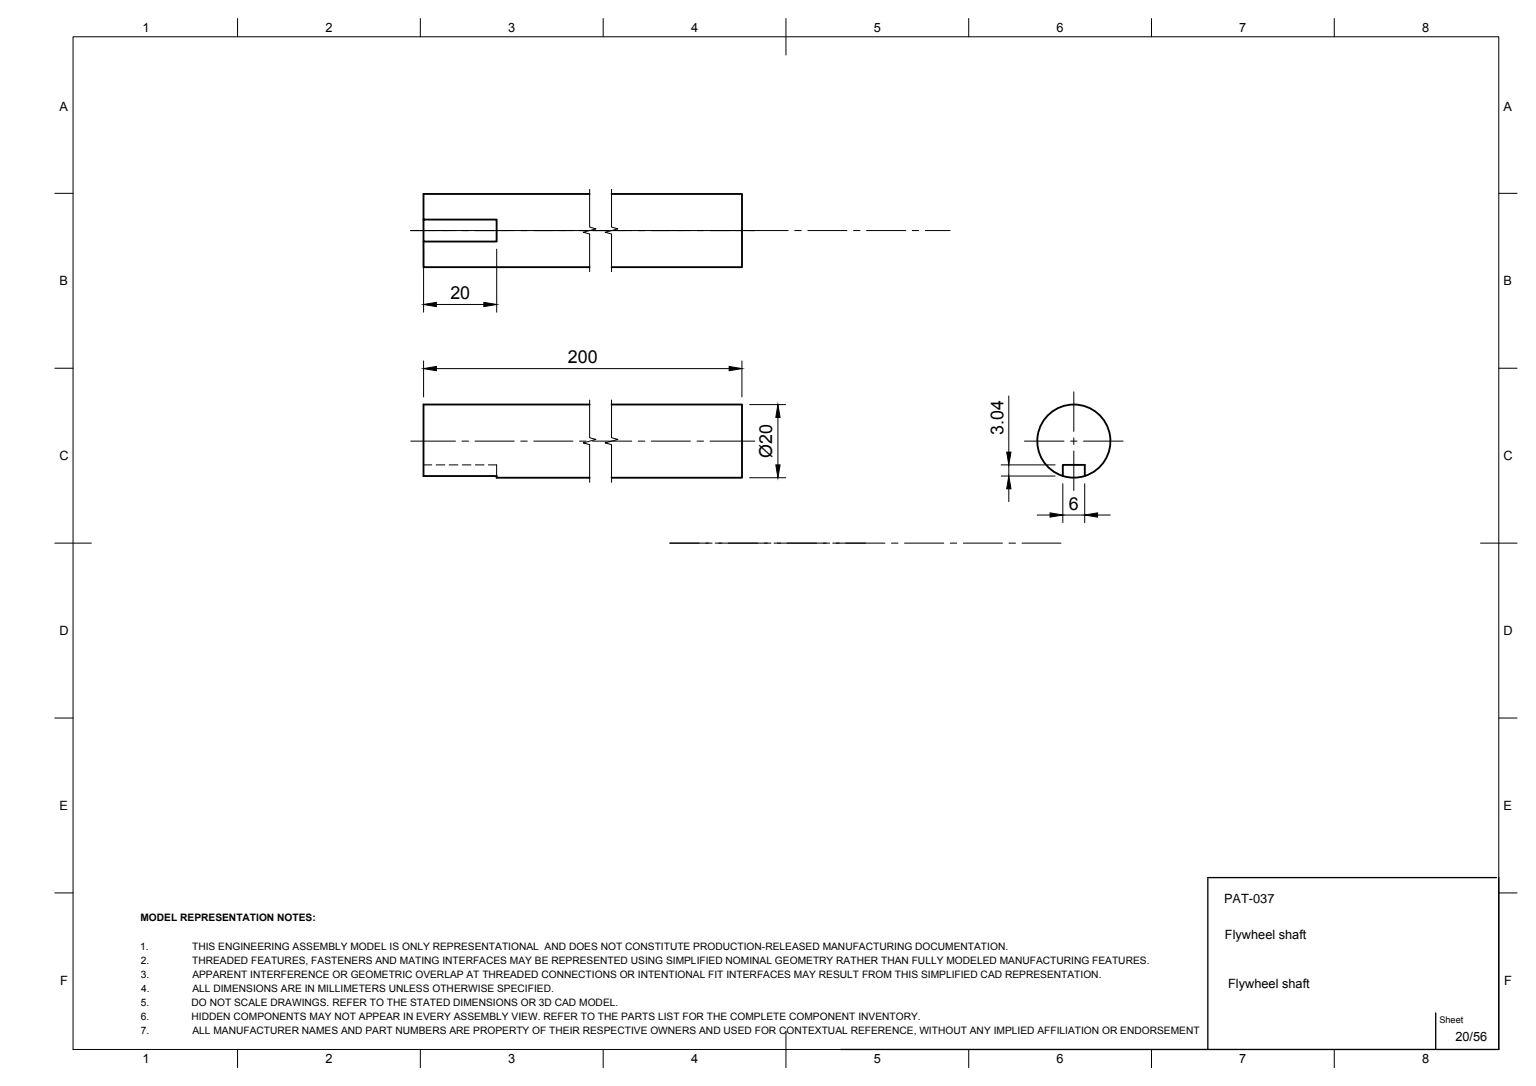
ISO-10303-21;
HEADER;
/* Generated by software containing ST-Developer
 * from STEP Tools, Inc. (www.steptools.com) 
 */

FILE_DESCRIPTION(
/* description */ ('Flywheel Crank-Slider'),
/* implementation_level */ '2;1');

FILE_NAME(
/* name */ 'Flywheel shaft.step',
/* time_stamp */ '2026-10-28T03:23:13-07:00',
/* author */ (''),
/* organization */ (''),
/* preprocessor_version */ 'ST-DEVELOPER v20.2',
/* originating_system */ 'Autodesk Translation Framework v15.17.0.0',
/* authorisation */ '');

FILE_SCHEMA (('AUTOMOTIVE_DESIGN { 1 0 10303 214 3 1 1 }'));
ENDSEC;

DATA;
#10=MECHANICAL_DESIGN_GEOMETRIC_PRESENTATION_REPRESENTATION('',(#690),#17322);
#585=SHAPE_REPRESENTATION_RELATIONSHIP('SRR','None',#17583,#637);
#637=ADVANCED_BREP_SHAPE_REPRESENTATION('',(#747),#17287);
#690=STYLED_ITEM('',(#17931),#747);
#747=MANIFOLD_SOLID_BREP('Body1',#9072);
#1175=PLANE('',#10186);
#1176=PLANE('',#10187);
#1177=PLANE('',#10189);
#1178=PLANE('',#10190);
#1179=PLANE('',#10195);
#1180=PLANE('',#10196);
#1595=FACE_OUTER_BOUND('',#2253,.T.);
#1596=FACE_OUTER_BOUND('',#2254,.T.);
#1597=FACE_OUTER_BOUND('',#2255,.T.);
#1598=FACE_OUTER_BOUND('',#2256,.T.);
#1599=FACE_OUTER_BOUND('',#2257,.T.);
#1600=FACE_OUTER_BOUND('',#2258,.T.);
#1601=FACE_OUTER_BOUND('',#2259,.T.);
#2253=EDGE_LOOP('',(#7278,#7279,#7280,#7281));
#2254=EDGE_LOOP('',(#7282,#7283,#7284,#7285));
#2255=EDGE_LOOP('',(#7286,#7287,#7288,#7289));
#2256=EDGE_LOOP('',(#7290,#7291,#7292,#7293));
#2257=EDGE_LOOP('',(#7294,#7295,#7296,#7297,#7298,#7299,#7300,#7301));
#2258=EDGE_LOOP('',(#7302,#7303,#7304,#7305,#7306));
#2259=EDGE_LOOP('',(#7307));
#2972=LINE('',#15405,#3583);
#2973=LINE('',#15407,#3584);
#2974=LINE('',#15409,#3585);
#2975=LINE('',#15410,#3586);
#2976=LINE('',#15415,#3587);
#2977=LINE('',#15416,#3588);
#2978=LINE('',#15419,#3589);
#2979=LINE('',#15421,#3590);
#2980=LINE('',#15422,#3591);
#2981=LINE('',#15424,#3592);
#2982=LINE('',#15429,#3593);
#3583=VECTOR('',#12190,1.);
#3584=VECTOR('',#12191,1.);
#3585=VECTOR('',#12192,1.);
#3586=VECTOR('',#12193,1.);
#3587=VECTOR('',#12198,1.);
#3588=VECTOR('',#12199,1.);
#3589=VECTOR('',#12202,1.);
#3590=VECTOR('',#12203,1.);
#3591=VECTOR('',#12204,1.);
#3592=VECTOR('',#12207,1.);
#3593=VECTOR('',#12212,1.);
#4036=CIRCLE('',#10188,1.);
#4037=CIRCLE('',#10192,1.);
#4038=CIRCLE('',#10193,1.);
#4039=CIRCLE('',#10194,1.);
#4659=VERTEX_POINT('',#15403);
#4660=VERTEX_POINT('',#15404);
#4661=VERTEX_POINT('',#15406);
#4662=VERTEX_POINT('',#15408);
#4663=VERTEX_POINT('',#15412);
#4664=VERTEX_POINT('',#15414);
#4665=VERTEX_POINT('',#15418);
#4666=VERTEX_POINT('',#15420);
#4667=VERTEX_POINT('',#15426);
#4668=VERTEX_POINT('',#15428);
#5596=EDGE_CURVE('',#4659,#4660,#2972,.T.);
#5597=EDGE_CURVE('',#4661,#4659,#2973,.T.);
#5598=EDGE_CURVE('',#4662,#4661,#2974,.T.);
#5599=EDGE_CURVE('',#4662,#4660,#2975,.T.);
#5600=EDGE_CURVE('',#4660,#4663,#4036,.T.);
#5601=EDGE_CURVE('',#4664,#4662,#2976,.T.);
#5602=EDGE_CURVE('',#4663,#4664,#2977,.T.);
#5603=EDGE_CURVE('',#4663,#4665,#2978,.T.);
#5604=EDGE_CURVE('',#4664,#4666,#2979,.T.);
#5605=EDGE_CURVE('',#4665,#4666,#2980,.T.);
#5606=EDGE_CURVE('',#4666,#4661,#2981,.T.);
#5607=EDGE_CURVE('',#4667,#4665,#4037,.T.);
#5608=EDGE_CURVE('',#4667,#4668,#2982,.T.);
#5609=EDGE_CURVE('',#4668,#4668,#4038,.T.);
#5610=EDGE_CURVE('',#4659,#4667,#4039,.T.);
#7278=ORIENTED_EDGE('',*,*,#5596,.F.);
#7279=ORIENTED_EDGE('',*,*,#5597,.F.);
#7280=ORIENTED_EDGE('',*,*,#5598,.F.);
#7281=ORIENTED_EDGE('',*,*,#5599,.T.);
#7282=ORIENTED_EDGE('',*,*,#5600,.F.);
#7283=ORIENTED_EDGE('',*,*,#5599,.F.);
#7284=ORIENTED_EDGE('',*,*,#5601,.F.);
#7285=ORIENTED_EDGE('',*,*,#5602,.F.);
#7286=ORIENTED_EDGE('',*,*,#5603,.F.);
#7287=ORIENTED_EDGE('',*,*,#5602,.T.);
#7288=ORIENTED_EDGE('',*,*,#5604,.T.);
#7289=ORIENTED_EDGE('',*,*,#5605,.F.);
#7290=ORIENTED_EDGE('',*,*,#5601,.T.);
#7291=ORIENTED_EDGE('',*,*,#5598,.T.);
#7292=ORIENTED_EDGE('',*,*,#5606,.F.);
#7293=ORIENTED_EDGE('',*,*,#5604,.F.);
#7294=ORIENTED_EDGE('',*,*,#5596,.T.);
#7295=ORIENTED_EDGE('',*,*,#5600,.T.);
#7296=ORIENTED_EDGE('',*,*,#5603,.T.);
#7297=ORIENTED_EDGE('',*,*,#5607,.F.);
#7298=ORIENTED_EDGE('',*,*,#5608,.T.);
#7299=ORIENTED_EDGE('',*,*,#5609,.T.);
#7300=ORIENTED_EDGE('',*,*,#5608,.F.);
#7301=ORIENTED_EDGE('',*,*,#5610,.F.);
#7302=ORIENTED_EDGE('',*,*,#5597,.T.);
#7303=ORIENTED_EDGE('',*,*,#5610,.T.);
#7304=ORIENTED_EDGE('',*,*,#5607,.T.);
#7305=ORIENTED_EDGE('',*,*,#5605,.T.);
#7306=ORIENTED_EDGE('',*,*,#5606,.T.);
#7307=ORIENTED_EDGE('',*,*,#5609,.F.);
#8423=CYLINDRICAL_SURFACE('',#10191,1.);
#8786=ADVANCED_FACE('',(#1595),#1175,.F.);
#8787=ADVANCED_FACE('',(#1596),#1176,.T.);
#8788=ADVANCED_FACE('',(#1597),#1177,.F.);
#8789=ADVANCED_FACE('',(#1598),#1178,.F.);
#8790=ADVANCED_FACE('',(#1599),#8423,.T.);
#8791=ADVANCED_FACE('',(#1600),#1179,.T.);
#8792=ADVANCED_FACE('',(#1601),#1180,.F.);
#9072=CLOSED_SHELL('',(#8786,#8787,#8788,#8789,#8790,#8791,#8792));
#10185=AXIS2_PLACEMENT_3D('',#15401,#12186,#12187);
#10186=AXIS2_PLACEMENT_3D('',#15402,#12188,#12189);
#10187=AXIS2_PLACEMENT_3D('',#15411,#12194,#12195);
#10188=AXIS2_PLACEMENT_3D('',#15413,#12196,#12197);
#10189=AXIS2_PLACEMENT_3D('',#15417,#12200,#12201);
#10190=AXIS2_PLACEMENT_3D('',#15423,#12205,#12206);
#10191=AXIS2_PLACEMENT_3D('',#15425,#12208,#12209);
#10192=AXIS2_PLACEMENT_3D('',#15427,#12210,#12211);
#10193=AXIS2_PLACEMENT_3D('',#15430,#12213,#12214);
#10194=AXIS2_PLACEMENT_3D('',#15431,#12215,#12216);
#10195=AXIS2_PLACEMENT_3D('',#15432,#12217,#12218);
#10196=AXIS2_PLACEMENT_3D('',#15433,#12219,#12220);
#12186=DIRECTION('axis',(0.,0.,1.));
#12187=DIRECTION('refdir',(1.,0.,0.));
#12188=DIRECTION('center_axis',(-1.,0.,0.));
#12189=DIRECTION('ref_axis',(0.,0.,1.));
#12190=DIRECTION('',(0.,-1.,0.));
#12191=DIRECTION('',(0.,0.,-1.));
#12192=DIRECTION('',(0.,1.,0.));
#12193=DIRECTION('',(0.,0.,-1.));
#12194=DIRECTION('center_axis',(0.,1.,0.));
#12195=DIRECTION('ref_axis',(1.,0.,0.));
#12196=DIRECTION('center_axis',(0.,-1.,0.));
#12197=DIRECTION('ref_axis',(1.,0.,0.));
#12198=DIRECTION('',(-1.,0.,0.));
#12199=DIRECTION('',(0.,0.,1.));
#12200=DIRECTION('center_axis',(1.,0.,0.));
#12201=DIRECTION('ref_axis',(0.,0.,-1.));
#12202=DIRECTION('',(0.,1.,0.));
#12203=DIRECTION('',(0.,1.,0.));
#12204=DIRECTION('',(0.,0.,1.));
#12205=DIRECTION('center_axis',(0.,0.,1.));
#12206=DIRECTION('ref_axis',(1.,0.,0.));
#12207=DIRECTION('',(-1.,0.,0.));
#12208=DIRECTION('center_axis',(0.,1.,0.));
#12209=DIRECTION('ref_axis',(1.,0.,0.));
#12210=DIRECTION('center_axis',(0.,1.,0.));
#12211=DIRECTION('ref_axis',(1.,0.,0.));
#12212=DIRECTION('',(0.,-1.,0.));
#12213=DIRECTION('center_axis',(0.,1.,0.));
#12214=DIRECTION('ref_axis',(1.,0.,0.));
#12215=DIRECTION('center_axis',(0.,1.,0.));
#12216=DIRECTION('ref_axis',(1.,0.,0.));
#12217=DIRECTION('center_axis',(0.,1.,0.));
#12218=DIRECTION('ref_axis',(1.,0.,0.));
#12219=DIRECTION('center_axis',(0.,1.,0.));
#12220=DIRECTION('ref_axis',(1.,0.,0.));
#15401=CARTESIAN_POINT('',(0.,0.,0.));
#15402=CARTESIAN_POINT('Origin',(-0.3,-1.,8.9));
#15403=CARTESIAN_POINT('',(-0.3,1.,9.04606079858305));
#15404=CARTESIAN_POINT('',(-0.3,-1.,9.04606079858305));
#15405=CARTESIAN_POINT('',(-0.3,-19.,9.04606079858305));
#15406=CARTESIAN_POINT('',(-0.3,1.,9.35));
#15407=CARTESIAN_POINT('',(-0.3,1.,9.45));
#15408=CARTESIAN_POINT('',(-0.3,-1.,9.35));
#15409=CARTESIAN_POINT('',(-0.3,-1.,9.35));
#15410=CARTESIAN_POINT('',(-0.3,-1.,9.35));
#15411=CARTESIAN_POINT('Origin',(0.,-1.,9.125));
#15412=CARTESIAN_POINT('',(0.3,-1.,9.04606079858305));
#15413=CARTESIAN_POINT('Origin',(0.,-1.,10.));
#15414=CARTESIAN_POINT('',(0.3,-1.,9.35));
#15415=CARTESIAN_POINT('',(0.3,-1.,9.35));
#15416=CARTESIAN_POINT('',(0.3,-1.,8.9));
#15417=CARTESIAN_POINT('Origin',(0.3,-1.,9.35));
#15418=CARTESIAN_POINT('',(0.3,1.,9.04606079858305));
#15419=CARTESIAN_POINT('',(0.3,-19.,9.04606079858305));
#15420=CARTESIAN_POINT('',(0.3,1.,9.35));
#15421=CARTESIAN_POINT('',(0.3,-1.,9.35));
#15422=CARTESIAN_POINT('',(0.3,1.,9.675));
#15423=CARTESIAN_POINT('Origin',(-0.3,-1.,9.35));
#15424=CARTESIAN_POINT('',(-0.15,1.,9.35));
#15425=CARTESIAN_POINT('Origin',(0.,-19.,10.));
#15426=CARTESIAN_POINT('',(-1.,1.,10.));
#15427=CARTESIAN_POINT('Origin',(0.,1.,10.));
#15428=CARTESIAN_POINT('',(-1.,-19.,10.));
#15429=CARTESIAN_POINT('',(-1.,-19.,10.));
#15430=CARTESIAN_POINT('Origin',(0.,-19.,10.));
#15431=CARTESIAN_POINT('Origin',(0.,1.,10.));
#15432=CARTESIAN_POINT('Origin',(0.,1.,10.));
#15433=CARTESIAN_POINT('Origin',(0.,-19.,10.));
#17226=UNCERTAINTY_MEASURE_WITH_UNIT(LENGTH_MEASURE(0.001),#17323,
'DISTANCE_ACCURACY_VALUE',
'Maximum model space distance between geometric entities at asserted c
onnectivities');
#17261=UNCERTAINTY_MEASURE_WITH_UNIT(LENGTH_MEASURE(0.001),#17323,
'DISTANCE_ACCURACY_VALUE',
'Maximum model space distance between geometric entities at asserted c
onnectivities');
#17287=(
GEOMETRIC_REPRESENTATION_CONTEXT(3)
GLOBAL_UNCERTAINTY_ASSIGNED_CONTEXT((#17226))
GLOBAL_UNIT_ASSIGNED_CONTEXT((#17323,#17325,#17326))
REPRESENTATION_CONTEXT('','3D')
);
#17322=(
GEOMETRIC_REPRESENTATION_CONTEXT(3)
GLOBAL_UNCERTAINTY_ASSIGNED_CONTEXT((#17261))
GLOBAL_UNIT_ASSIGNED_CONTEXT((#17323,#17325,#17326))
REPRESENTATION_CONTEXT('','3D')
);
#17323=(
LENGTH_UNIT()
NAMED_UNIT(*)
SI_UNIT(.CENTI.,.METRE.)
);
#17325=(
NAMED_UNIT(*)
PLANE_ANGLE_UNIT()
SI_UNIT($,.RADIAN.)
);
#17326=(
NAMED_UNIT(*)
SI_UNIT($,.STERADIAN.)
SOLID_ANGLE_UNIT()
);
#17352=SHAPE_DEFINITION_REPRESENTATION(#17414,#17583);
#17414=PRODUCT_DEFINITION_SHAPE('',$,#17644);
#17583=SHAPE_REPRESENTATION('',(#10185),#17287);
#17618=PRODUCT_DEFINITION_CONTEXT('part definition',#17800,'design');
#17644=PRODUCT_DEFINITION('Flywheel shaft','Flywheel shaft',#17704,#17618);
#17704=PRODUCT_DEFINITION_FORMATION('',$,#17827);
#17800=APPLICATION_CONTEXT(
'Core Data for Automotive Mechanical Design Process');
#17801=PRODUCT_CONTEXT('part definition',#17800,'mechanical');
#17827=PRODUCT('Flywheel shaft','Flywheel shaft','Flywheel shaft',(#17801));
#17925=COLOUR_RGB('Grey',0.48,0.52,0.57);
#17926=FILL_AREA_STYLE_COLOUR('',#17925);
#17927=FILL_AREA_STYLE('',(#17926));
#17928=SURFACE_STYLE_FILL_AREA(#17927);
#17929=SURFACE_SIDE_STYLE('',(#17928));
#17930=SURFACE_STYLE_USAGE(.BOTH.,#17929);
#17931=PRESENTATION_STYLE_ASSIGNMENT((#17930));
ENDSEC;
END-ISO-10303-21;
